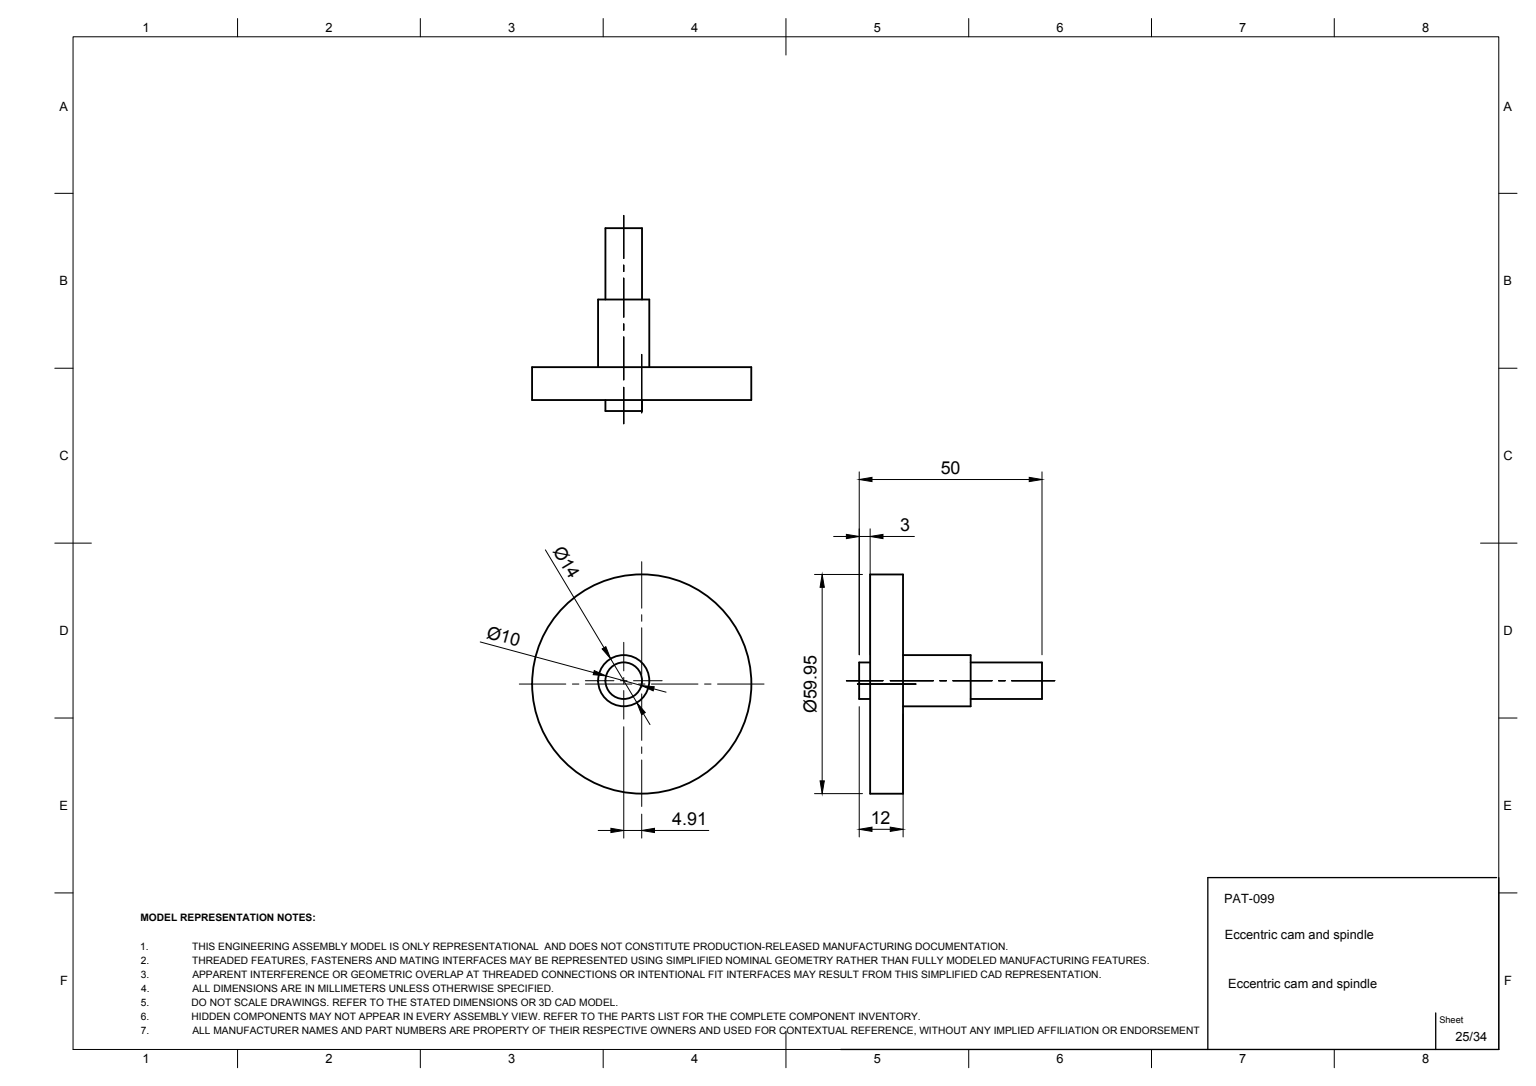
ISO-10303-21;
HEADER;
/* Generated by software containing ST-Developer
 * from STEP Tools, Inc. (www.steptools.com) 
 */

FILE_DESCRIPTION(
/* description */ ('PAT-099'),
/* implementation_level */ '2;1');

FILE_NAME(
/* name */ 'Eccentric cam and spindle.step',
/* time_stamp */ '2026-10-29T17:25:42-07:00',
/* author */ (''),
/* organization */ (''),
/* preprocessor_version */ 'ST-DEVELOPER v20.2',
/* originating_system */ 'Autodesk Translation Framework v15.17.0.0',
/* authorisation */ '');

FILE_SCHEMA (('AUTOMOTIVE_DESIGN { 1 0 10303 214 3 1 1 }'));
ENDSEC;

DATA;
#10=MECHANICAL_DESIGN_GEOMETRIC_PRESENTATION_REPRESENTATION('',(#347),#11035);
#297=SHAPE_REPRESENTATION_RELATIONSHIP('SRR','None',#11167,#322);
#322=ADVANCED_BREP_SHAPE_REPRESENTATION('',(#379),#11017);
#347=STYLED_ITEM('',(#11379),#379);
#379=MANIFOLD_SOLID_BREP('Body1',#4716);
#490=FACE_BOUND('',#1176,.T.);
#491=FACE_BOUND('',#1178,.T.);
#492=FACE_BOUND('',#1181,.T.);
#590=PLANE('',#5337);
#591=PLANE('',#5340);
#592=PLANE('',#5344);
#593=PLANE('',#5352);
#594=PLANE('',#5353);
#805=FACE_OUTER_BOUND('',#1175,.T.);
#806=FACE_OUTER_BOUND('',#1177,.T.);
#807=FACE_OUTER_BOUND('',#1179,.T.);
#808=FACE_OUTER_BOUND('',#1180,.T.);
#809=FACE_OUTER_BOUND('',#1182,.T.);
#810=FACE_OUTER_BOUND('',#1183,.T.);
#811=FACE_OUTER_BOUND('',#1184,.T.);
#812=FACE_OUTER_BOUND('',#1185,.T.);
#813=FACE_OUTER_BOUND('',#1186,.T.);
#1175=EDGE_LOOP('',(#3779));
#1176=EDGE_LOOP('',(#3780));
#1177=EDGE_LOOP('',(#3781));
#1178=EDGE_LOOP('',(#3782));
#1179=EDGE_LOOP('',(#3783,#3784,#3785,#3786));
#1180=EDGE_LOOP('',(#3787));
#1181=EDGE_LOOP('',(#3788));
#1182=EDGE_LOOP('',(#3789,#3790,#3791,#3792));
#1183=EDGE_LOOP('',(#3793,#3794,#3795,#3796));
#1184=EDGE_LOOP('',(#3797,#3798,#3799,#3800));
#1185=EDGE_LOOP('',(#3801));
#1186=EDGE_LOOP('',(#3802));
#1485=LINE('',#9933,#1737);
#1486=LINE('',#9940,#1738);
#1487=LINE('',#9943,#1739);
#1488=LINE('',#9948,#1740);
#1737=VECTOR('',#6466,2.99742622740447);
#1738=VECTOR('',#6475,0.7);
#1739=VECTOR('',#6478,0.5);
#1740=VECTOR('',#6485,0.5);
#2006=CIRCLE('',#5338,2.99742622740447);
#2007=CIRCLE('',#5339,0.5);
#2008=CIRCLE('',#5341,2.99742622740447);
#2009=CIRCLE('',#5342,0.7);
#2010=CIRCLE('',#5345,0.7);
#2011=CIRCLE('',#5346,0.5);
#2012=CIRCLE('',#5349,0.5);
#2013=CIRCLE('',#5351,0.5);
#2357=VERTEX_POINT('',#9923);
#2358=VERTEX_POINT('',#9925);
#2359=VERTEX_POINT('',#9928);
#2360=VERTEX_POINT('',#9930);
#2361=VERTEX_POINT('',#9935);
#2362=VERTEX_POINT('',#9937);
#2363=VERTEX_POINT('',#9942);
#2364=VERTEX_POINT('',#9946);
#2866=EDGE_CURVE('',#2357,#2357,#2006,.T.);
#2867=EDGE_CURVE('',#2358,#2358,#2007,.T.);
#2868=EDGE_CURVE('',#2359,#2359,#2008,.T.);
#2869=EDGE_CURVE('',#2360,#2360,#2009,.T.);
#2870=EDGE_CURVE('',#2357,#2359,#1485,.T.);
#2871=EDGE_CURVE('',#2361,#2361,#2010,.T.);
#2872=EDGE_CURVE('',#2362,#2362,#2011,.T.);
#2873=EDGE_CURVE('',#2360,#2361,#1486,.T.);
#2874=EDGE_CURVE('',#2362,#2363,#1487,.T.);
#2875=EDGE_CURVE('',#2363,#2363,#2012,.T.);
#2876=EDGE_CURVE('',#2364,#2364,#2013,.T.);
#2877=EDGE_CURVE('',#2364,#2358,#1488,.T.);
#3779=ORIENTED_EDGE('',*,*,#2866,.T.);
#3780=ORIENTED_EDGE('',*,*,#2867,.F.);
#3781=ORIENTED_EDGE('',*,*,#2868,.F.);
#3782=ORIENTED_EDGE('',*,*,#2869,.T.);
#3783=ORIENTED_EDGE('',*,*,#2866,.F.);
#3784=ORIENTED_EDGE('',*,*,#2870,.T.);
#3785=ORIENTED_EDGE('',*,*,#2868,.T.);
#3786=ORIENTED_EDGE('',*,*,#2870,.F.);
#3787=ORIENTED_EDGE('',*,*,#2871,.F.);
#3788=ORIENTED_EDGE('',*,*,#2872,.F.);
#3789=ORIENTED_EDGE('',*,*,#2869,.F.);
#3790=ORIENTED_EDGE('',*,*,#2873,.T.);
#3791=ORIENTED_EDGE('',*,*,#2871,.T.);
#3792=ORIENTED_EDGE('',*,*,#2873,.F.);
#3793=ORIENTED_EDGE('',*,*,#2872,.T.);
#3794=ORIENTED_EDGE('',*,*,#2874,.T.);
#3795=ORIENTED_EDGE('',*,*,#2875,.T.);
#3796=ORIENTED_EDGE('',*,*,#2874,.F.);
#3797=ORIENTED_EDGE('',*,*,#2876,.F.);
#3798=ORIENTED_EDGE('',*,*,#2877,.T.);
#3799=ORIENTED_EDGE('',*,*,#2867,.T.);
#3800=ORIENTED_EDGE('',*,*,#2877,.F.);
#3801=ORIENTED_EDGE('',*,*,#2876,.T.);
#3802=ORIENTED_EDGE('',*,*,#2875,.F.);
#4384=CYLINDRICAL_SURFACE('',#5343,2.99742622740447);
#4385=CYLINDRICAL_SURFACE('',#5347,0.7);
#4386=CYLINDRICAL_SURFACE('',#5348,0.5);
#4387=CYLINDRICAL_SURFACE('',#5350,0.5);
#4570=ADVANCED_FACE('',(#805,#490),#590,.T.);
#4571=ADVANCED_FACE('',(#806,#491),#591,.F.);
#4572=ADVANCED_FACE('',(#807),#4384,.T.);
#4573=ADVANCED_FACE('',(#808,#492),#592,.F.);
#4574=ADVANCED_FACE('',(#809),#4385,.T.);
#4575=ADVANCED_FACE('',(#810),#4386,.T.);
#4576=ADVANCED_FACE('',(#811),#4387,.T.);
#4577=ADVANCED_FACE('',(#812),#593,.T.);
#4578=ADVANCED_FACE('',(#813),#594,.F.);
#4716=CLOSED_SHELL('',(#4570,#4571,#4572,#4573,#4574,#4575,#4576,#4577,
#4578));
#5336=AXIS2_PLACEMENT_3D('',#9921,#6450,#6451);
#5337=AXIS2_PLACEMENT_3D('',#9922,#6452,#6453);
#5338=AXIS2_PLACEMENT_3D('',#9924,#6454,#6455);
#5339=AXIS2_PLACEMENT_3D('',#9926,#6456,#6457);
#5340=AXIS2_PLACEMENT_3D('',#9927,#6458,#6459);
#5341=AXIS2_PLACEMENT_3D('',#9929,#6460,#6461);
#5342=AXIS2_PLACEMENT_3D('',#9931,#6462,#6463);
#5343=AXIS2_PLACEMENT_3D('',#9932,#6464,#6465);
#5344=AXIS2_PLACEMENT_3D('',#9934,#6467,#6468);
#5345=AXIS2_PLACEMENT_3D('',#9936,#6469,#6470);
#5346=AXIS2_PLACEMENT_3D('',#9938,#6471,#6472);
#5347=AXIS2_PLACEMENT_3D('',#9939,#6473,#6474);
#5348=AXIS2_PLACEMENT_3D('',#9941,#6476,#6477);
#5349=AXIS2_PLACEMENT_3D('',#9944,#6479,#6480);
#5350=AXIS2_PLACEMENT_3D('',#9945,#6481,#6482);
#5351=AXIS2_PLACEMENT_3D('',#9947,#6483,#6484);
#5352=AXIS2_PLACEMENT_3D('',#9949,#6486,#6487);
#5353=AXIS2_PLACEMENT_3D('',#9950,#6488,#6489);
#6450=DIRECTION('axis',(0.,0.,1.));
#6451=DIRECTION('refdir',(1.,0.,0.));
#6452=DIRECTION('center_axis',(0.,0.,1.));
#6453=DIRECTION('ref_axis',(1.,0.,0.));
#6454=DIRECTION('center_axis',(0.,0.,1.));
#6455=DIRECTION('ref_axis',(1.,0.,0.));
#6456=DIRECTION('center_axis',(0.,0.,1.));
#6457=DIRECTION('ref_axis',(1.,0.,0.));
#6458=DIRECTION('center_axis',(0.,0.,1.));
#6459=DIRECTION('ref_axis',(1.,0.,0.));
#6460=DIRECTION('center_axis',(0.,0.,1.));
#6461=DIRECTION('ref_axis',(1.,0.,0.));
#6462=DIRECTION('center_axis',(0.,0.,1.));
#6463=DIRECTION('ref_axis',(1.,0.,0.));
#6464=DIRECTION('center_axis',(0.,0.,1.));
#6465=DIRECTION('ref_axis',(1.,0.,0.));
#6466=DIRECTION('',(0.,0.,-1.));
#6467=DIRECTION('center_axis',(0.,0.,1.));
#6468=DIRECTION('ref_axis',(1.,0.,0.));
#6469=DIRECTION('center_axis',(0.,0.,1.));
#6470=DIRECTION('ref_axis',(1.,0.,0.));
#6471=DIRECTION('center_axis',(0.,0.,-1.));
#6472=DIRECTION('ref_axis',(1.,0.,0.));
#6473=DIRECTION('center_axis',(0.,0.,1.));
#6474=DIRECTION('ref_axis',(1.,0.,0.));
#6475=DIRECTION('',(0.,0.,-1.));
#6476=DIRECTION('center_axis',(0.,0.,1.));
#6477=DIRECTION('ref_axis',(1.,0.,0.));
#6478=DIRECTION('',(0.,0.,-1.));
#6479=DIRECTION('center_axis',(0.,0.,1.));
#6480=DIRECTION('ref_axis',(1.,0.,0.));
#6481=DIRECTION('center_axis',(0.,0.,1.));
#6482=DIRECTION('ref_axis',(1.,0.,0.));
#6483=DIRECTION('center_axis',(0.,0.,1.));
#6484=DIRECTION('ref_axis',(1.,0.,0.));
#6485=DIRECTION('',(0.,0.,-1.));
#6486=DIRECTION('center_axis',(0.,0.,1.));
#6487=DIRECTION('ref_axis',(1.,0.,0.));
#6488=DIRECTION('center_axis',(0.,0.,1.));
#6489=DIRECTION('ref_axis',(1.,0.,0.));
#9921=CARTESIAN_POINT('',(0.,0.,0.));
#9922=CARTESIAN_POINT('Origin',(0.5,0.,5.7));
#9923=CARTESIAN_POINT('',(-2.49742622740447,-3.67078843507121E-16,5.7));
#9924=CARTESIAN_POINT('Origin',(0.5,0.,5.7));
#9925=CARTESIAN_POINT('',(-0.5,-6.12323399573677E-17,5.7));
#9926=CARTESIAN_POINT('Origin',(0.,0.,5.7));
#9927=CARTESIAN_POINT('Origin',(0.5,0.,4.8));
#9928=CARTESIAN_POINT('',(-2.49742622740447,-3.67078843507121E-16,4.8));
#9929=CARTESIAN_POINT('Origin',(0.5,0.,4.8));
#9930=CARTESIAN_POINT('',(-0.7,-8.57252759403147E-17,4.8));
#9931=CARTESIAN_POINT('Origin',(0.,0.,4.8));
#9932=CARTESIAN_POINT('Origin',(0.5,0.,4.8));
#9933=CARTESIAN_POINT('',(-2.49742622740447,-3.67078843507121E-16,4.8));
#9934=CARTESIAN_POINT('Origin',(0.,0.,2.95));
#9935=CARTESIAN_POINT('',(-0.7,-8.57252759403147E-17,2.95));
#9936=CARTESIAN_POINT('Origin',(0.,0.,2.95));
#9937=CARTESIAN_POINT('',(-0.5,6.12323399573677E-17,2.95));
#9938=CARTESIAN_POINT('Origin',(0.,0.,2.95));
#9939=CARTESIAN_POINT('Origin',(0.,0.,2.95));
#9940=CARTESIAN_POINT('',(-0.7,-8.57252759403147E-17,2.95));
#9941=CARTESIAN_POINT('Origin',(0.,0.,1.));
#9942=CARTESIAN_POINT('',(-0.5,-6.12323399573677E-17,1.));
#9943=CARTESIAN_POINT('',(-0.5,-6.12323399573677E-17,1.));
#9944=CARTESIAN_POINT('Origin',(0.,0.,1.));
#9945=CARTESIAN_POINT('Origin',(0.,0.,1.));
#9946=CARTESIAN_POINT('',(-0.5,-6.12323399573677E-17,6.));
#9947=CARTESIAN_POINT('Origin',(0.,0.,6.));
#9948=CARTESIAN_POINT('',(-0.5,-6.12323399573677E-17,1.));
#9949=CARTESIAN_POINT('Origin',(0.,0.,6.));
#9950=CARTESIAN_POINT('Origin',(0.,0.,1.));
#10984=UNCERTAINTY_MEASURE_WITH_UNIT(LENGTH_MEASURE(0.001),#11036,
'DISTANCE_ACCURACY_VALUE',
'Maximum model space distance between geometric entities at asserted c
onnectivities');
#11002=UNCERTAINTY_MEASURE_WITH_UNIT(LENGTH_MEASURE(0.001),#11036,
'DISTANCE_ACCURACY_VALUE',
'Maximum model space distance between geometric entities at asserted c
onnectivities');
#11017=(
GEOMETRIC_REPRESENTATION_CONTEXT(3)
GLOBAL_UNCERTAINTY_ASSIGNED_CONTEXT((#10984))
GLOBAL_UNIT_ASSIGNED_CONTEXT((#11036,#11038,#11039))
REPRESENTATION_CONTEXT('','3D')
);
#11035=(
GEOMETRIC_REPRESENTATION_CONTEXT(3)
GLOBAL_UNCERTAINTY_ASSIGNED_CONTEXT((#11002))
GLOBAL_UNIT_ASSIGNED_CONTEXT((#11036,#11038,#11039))
REPRESENTATION_CONTEXT('','3D')
);
#11036=(
LENGTH_UNIT()
NAMED_UNIT(*)
SI_UNIT(.CENTI.,.METRE.)
);
#11038=(
NAMED_UNIT(*)
PLANE_ANGLE_UNIT()
SI_UNIT($,.RADIAN.)
);
#11039=(
NAMED_UNIT(*)
SI_UNIT($,.STERADIAN.)
SOLID_ANGLE_UNIT()
);
#11054=SHAPE_DEFINITION_REPRESENTATION(#11088,#11167);
#11088=PRODUCT_DEFINITION_SHAPE('',$,#11200);
#11167=SHAPE_REPRESENTATION('',(#5336),#11017);
#11185=PRODUCT_DEFINITION_CONTEXT('part definition',#11283,'design');
#11200=PRODUCT_DEFINITION('Eccentric cam and spindle',
'Eccentric cam and spindle',#11232,#11185);
#11232=PRODUCT_DEFINITION_FORMATION('',$,#11299);
#11283=APPLICATION_CONTEXT(
'Core Data for Automotive Mechanical Design Process');
#11284=PRODUCT_CONTEXT('part definition',#11283,'mechanical');
#11299=PRODUCT('Eccentric cam and spindle','Eccentric cam and spindle',
'Eccentric cam and spindle',(#11284));
#11373=COLOUR_RGB('Sky Blue',0.24,0.69,0.87);
#11374=FILL_AREA_STYLE_COLOUR('',#11373);
#11375=FILL_AREA_STYLE('',(#11374));
#11376=SURFACE_STYLE_FILL_AREA(#11375);
#11377=SURFACE_SIDE_STYLE('',(#11376));
#11378=SURFACE_STYLE_USAGE(.BOTH.,#11377);
#11379=PRESENTATION_STYLE_ASSIGNMENT((#11378));
ENDSEC;
END-ISO-10303-21;
